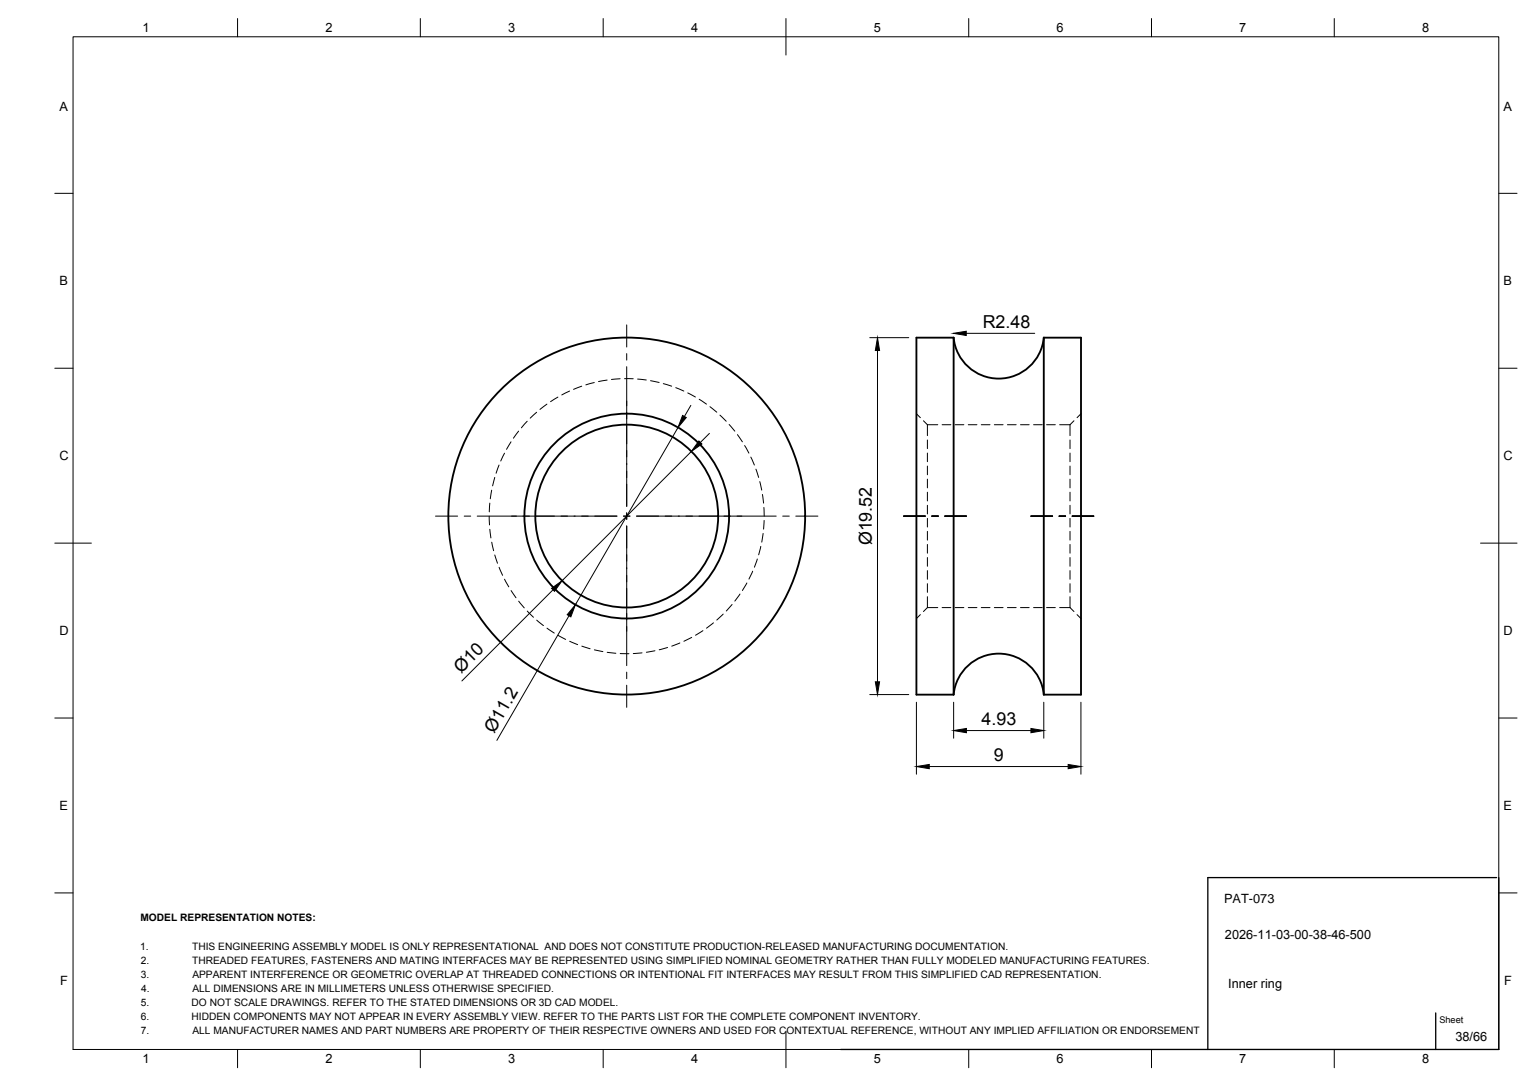
ISO-10303-21;
HEADER;
/* Generated by software containing ST-Developer
 * from STEP Tools, Inc. (www.steptools.com) 
 */

FILE_DESCRIPTION(
/* description */ ('Manual piston pump'),
/* implementation_level */ '2;1');

FILE_NAME(
/* name */ 'Inner ring.step',
/* time_stamp */ '2026-11-02T16:54:23-08:00',
/* author */ (''),
/* organization */ (''),
/* preprocessor_version */ 'ST-DEVELOPER v20.2',
/* originating_system */ 'Autodesk Translation Framework v15.17.0.0',
/* authorisation */ '');

FILE_SCHEMA (('AUTOMOTIVE_DESIGN { 1 0 10303 214 3 1 1 }'));
ENDSEC;

DATA;
#10=MECHANICAL_DESIGN_GEOMETRIC_PRESENTATION_REPRESENTATION('',(#711),#19043);
#537=CONICAL_SURFACE('',#10717,0.53,0.785398163397448);
#538=CONICAL_SURFACE('',#10724,0.53,0.785398163397448);
#559=TOROIDAL_SURFACE('',#10706,1.,0.247676);
#585=SHAPE_REPRESENTATION_RELATIONSHIP('SRR','None',#19332,#648);
#648=ADVANCED_BREP_SHAPE_REPRESENTATION('',(#781),#18999);
#711=STYLED_ITEM('',(#19664),#781);
#781=MANIFOLD_SOLID_BREP('Body1',#9497);
#946=FACE_BOUND('',#2229,.T.);
#947=FACE_BOUND('',#2232,.T.);
#1183=CYLINDRICAL_SURFACE('',#10712,0.976185);
#1184=CYLINDRICAL_SURFACE('',#10714,0.5);
#1185=CYLINDRICAL_SURFACE('',#10720,0.976185);
#1530=FACE_OUTER_BOUND('',#2224,.T.);
#1531=FACE_OUTER_BOUND('',#2225,.T.);
#1532=FACE_OUTER_BOUND('',#2226,.T.);
#1533=FACE_OUTER_BOUND('',#2227,.T.);
#1534=FACE_OUTER_BOUND('',#2228,.T.);
#1535=FACE_OUTER_BOUND('',#2230,.T.);
#1536=FACE_OUTER_BOUND('',#2231,.T.);
#1537=FACE_OUTER_BOUND('',#2233,.T.);
#2224=EDGE_LOOP('',(#7249,#7250,#7251,#7252,#7253,#7254));
#2225=EDGE_LOOP('',(#7255,#7256,#7257,#7258,#7259));
#2226=EDGE_LOOP('',(#7260,#7261,#7262,#7263));
#2227=EDGE_LOOP('',(#7264,#7265,#7266,#7267));
#2228=EDGE_LOOP('',(#7268));
#2229=EDGE_LOOP('',(#7269));
#2230=EDGE_LOOP('',(#7270,#7271,#7272,#7273,#7274));
#2231=EDGE_LOOP('',(#7275));
#2232=EDGE_LOOP('',(#7276));
#2233=EDGE_LOOP('',(#7277,#7278,#7279,#7280));
#2861=CIRCLE('',#10707,0.976185);
#2862=CIRCLE('',#10708,0.976185);
#2863=CIRCLE('',#10709,0.247676);
#2864=CIRCLE('',#10710,0.976185);
#2865=CIRCLE('',#10711,0.976185);
#2866=CIRCLE('',#10713,0.976185);
#2867=CIRCLE('',#10715,0.5);
#2868=CIRCLE('',#10716,0.5);
#2869=CIRCLE('',#10718,0.56);
#2870=CIRCLE('',#10721,0.976185);
#2871=CIRCLE('',#10723,0.56);
#3422=LINE('',#15764,#4026);
#3423=LINE('',#15770,#4027);
#3424=LINE('',#15774,#4028);
#3425=LINE('',#15780,#4029);
#3426=LINE('',#15785,#4030);
#4026=VECTOR('',#12710,0.976185);
#4027=VECTOR('',#12717,0.5);
#4028=VECTOR('',#12722,0.53);
#4029=VECTOR('',#12731,0.976185);
#4030=VECTOR('',#12738,0.53);
#4676=VERTEX_POINT('',#15753);
#4677=VERTEX_POINT('',#15754);
#4678=VERTEX_POINT('',#15757);
#4679=VERTEX_POINT('',#15759);
#4680=VERTEX_POINT('',#15763);
#4681=VERTEX_POINT('',#15767);
#4682=VERTEX_POINT('',#15769);
#4683=VERTEX_POINT('',#15773);
#4684=VERTEX_POINT('',#15778);
#4685=VERTEX_POINT('',#15782);
#5611=EDGE_CURVE('',#4676,#4677,#2861,.T.);
#5612=EDGE_CURVE('',#4677,#4676,#2862,.T.);
#5613=EDGE_CURVE('',#4677,#4678,#2863,.T.);
#5614=EDGE_CURVE('',#4679,#4678,#2864,.T.);
#5615=EDGE_CURVE('',#4678,#4679,#2865,.T.);
#5616=EDGE_CURVE('',#4679,#4680,#3422,.T.);
#5617=EDGE_CURVE('',#4680,#4680,#2866,.T.);
#5618=EDGE_CURVE('',#4681,#4681,#2867,.T.);
#5619=EDGE_CURVE('',#4681,#4682,#3423,.T.);
#5620=EDGE_CURVE('',#4682,#4682,#2868,.T.);
#5621=EDGE_CURVE('',#4682,#4683,#3424,.T.);
#5622=EDGE_CURVE('',#4683,#4683,#2869,.T.);
#5623=EDGE_CURVE('',#4684,#4684,#2870,.T.);
#5624=EDGE_CURVE('',#4684,#4676,#3425,.T.);
#5625=EDGE_CURVE('',#4685,#4685,#2871,.T.);
#5626=EDGE_CURVE('',#4685,#4681,#3426,.T.);
#7249=ORIENTED_EDGE('',*,*,#5611,.F.);
#7250=ORIENTED_EDGE('',*,*,#5612,.F.);
#7251=ORIENTED_EDGE('',*,*,#5613,.T.);
#7252=ORIENTED_EDGE('',*,*,#5614,.F.);
#7253=ORIENTED_EDGE('',*,*,#5615,.F.);
#7254=ORIENTED_EDGE('',*,*,#5613,.F.);
#7255=ORIENTED_EDGE('',*,*,#5614,.T.);
#7256=ORIENTED_EDGE('',*,*,#5615,.T.);
#7257=ORIENTED_EDGE('',*,*,#5616,.T.);
#7258=ORIENTED_EDGE('',*,*,#5617,.T.);
#7259=ORIENTED_EDGE('',*,*,#5616,.F.);
#7260=ORIENTED_EDGE('',*,*,#5618,.T.);
#7261=ORIENTED_EDGE('',*,*,#5619,.T.);
#7262=ORIENTED_EDGE('',*,*,#5620,.F.);
#7263=ORIENTED_EDGE('',*,*,#5619,.F.);
#7264=ORIENTED_EDGE('',*,*,#5620,.T.);
#7265=ORIENTED_EDGE('',*,*,#5621,.T.);
#7266=ORIENTED_EDGE('',*,*,#5622,.F.);
#7267=ORIENTED_EDGE('',*,*,#5621,.F.);
#7268=ORIENTED_EDGE('',*,*,#5617,.F.);
#7269=ORIENTED_EDGE('',*,*,#5622,.T.);
#7270=ORIENTED_EDGE('',*,*,#5623,.F.);
#7271=ORIENTED_EDGE('',*,*,#5624,.T.);
#7272=ORIENTED_EDGE('',*,*,#5611,.T.);
#7273=ORIENTED_EDGE('',*,*,#5612,.T.);
#7274=ORIENTED_EDGE('',*,*,#5624,.F.);
#7275=ORIENTED_EDGE('',*,*,#5623,.T.);
#7276=ORIENTED_EDGE('',*,*,#5625,.F.);
#7277=ORIENTED_EDGE('',*,*,#5625,.T.);
#7278=ORIENTED_EDGE('',*,*,#5626,.T.);
#7279=ORIENTED_EDGE('',*,*,#5618,.F.);
#7280=ORIENTED_EDGE('',*,*,#5626,.F.);
#8708=PLANE('',#10719);
#8709=PLANE('',#10722);
#9135=ADVANCED_FACE('',(#1530),#559,.F.);
#9136=ADVANCED_FACE('',(#1531),#1183,.T.);
#9137=ADVANCED_FACE('',(#1532),#1184,.F.);
#9138=ADVANCED_FACE('',(#1533),#537,.F.);
#9139=ADVANCED_FACE('',(#1534,#946),#8708,.T.);
#9140=ADVANCED_FACE('',(#1535),#1185,.T.);
#9141=ADVANCED_FACE('',(#1536,#947),#8709,.T.);
#9142=ADVANCED_FACE('',(#1537),#538,.F.);
#9497=CLOSED_SHELL('',(#9135,#9136,#9137,#9138,#9139,#9140,#9141,#9142));
#10705=AXIS2_PLACEMENT_3D('',#15751,#12694,#12695);
#10706=AXIS2_PLACEMENT_3D('',#15752,#12696,#12697);
#10707=AXIS2_PLACEMENT_3D('',#15755,#12698,#12699);
#10708=AXIS2_PLACEMENT_3D('',#15756,#12700,#12701);
#10709=AXIS2_PLACEMENT_3D('',#15758,#12702,#12703);
#10710=AXIS2_PLACEMENT_3D('',#15760,#12704,#12705);
#10711=AXIS2_PLACEMENT_3D('',#15761,#12706,#12707);
#10712=AXIS2_PLACEMENT_3D('',#15762,#12708,#12709);
#10713=AXIS2_PLACEMENT_3D('',#15765,#12711,#12712);
#10714=AXIS2_PLACEMENT_3D('',#15766,#12713,#12714);
#10715=AXIS2_PLACEMENT_3D('',#15768,#12715,#12716);
#10716=AXIS2_PLACEMENT_3D('',#15771,#12718,#12719);
#10717=AXIS2_PLACEMENT_3D('',#15772,#12720,#12721);
#10718=AXIS2_PLACEMENT_3D('',#15775,#12723,#12724);
#10719=AXIS2_PLACEMENT_3D('',#15776,#12725,#12726);
#10720=AXIS2_PLACEMENT_3D('',#15777,#12727,#12728);
#10721=AXIS2_PLACEMENT_3D('',#15779,#12729,#12730);
#10722=AXIS2_PLACEMENT_3D('',#15781,#12732,#12733);
#10723=AXIS2_PLACEMENT_3D('',#15783,#12734,#12735);
#10724=AXIS2_PLACEMENT_3D('',#15784,#12736,#12737);
#12694=DIRECTION('axis',(0.,0.,1.));
#12695=DIRECTION('refdir',(1.,0.,0.));
#12696=DIRECTION('center_axis',(0.,-1.,0.));
#12697=DIRECTION('ref_axis',(0.,0.,-1.));
#12698=DIRECTION('center_axis',(0.,-1.,0.));
#12699=DIRECTION('ref_axis',(1.,0.,0.));
#12700=DIRECTION('center_axis',(0.,-1.,0.));
#12701=DIRECTION('ref_axis',(1.,0.,0.));
#12702=DIRECTION('center_axis',(1.,0.,1.22464679914735E-16));
#12703=DIRECTION('ref_axis',(-1.22464679914735E-16,0.,1.));
#12704=DIRECTION('center_axis',(0.,1.,0.));
#12705=DIRECTION('ref_axis',(1.,0.,0.));
#12706=DIRECTION('center_axis',(0.,1.,0.));
#12707=DIRECTION('ref_axis',(1.,0.,0.));
#12708=DIRECTION('center_axis',(0.,-1.,0.));
#12709=DIRECTION('ref_axis',(1.,0.,0.));
#12710=DIRECTION('',(0.,1.,0.));
#12711=DIRECTION('center_axis',(0.,-1.,0.));
#12712=DIRECTION('ref_axis',(1.,0.,0.));
#12713=DIRECTION('center_axis',(0.,-1.,0.));
#12714=DIRECTION('ref_axis',(1.,0.,0.));
#12715=DIRECTION('center_axis',(0.,-1.,0.));
#12716=DIRECTION('ref_axis',(1.,0.,0.));
#12717=DIRECTION('',(0.,1.,0.));
#12718=DIRECTION('center_axis',(0.,-1.,0.));
#12719=DIRECTION('ref_axis',(1.,0.,0.));
#12720=DIRECTION('center_axis',(0.,1.,0.));
#12721=DIRECTION('ref_axis',(1.,0.,0.));
#12722=DIRECTION('',(-0.707106781186547,0.707106781186548,-8.65956056235493E-17));
#12723=DIRECTION('center_axis',(0.,-1.,0.));
#12724=DIRECTION('ref_axis',(1.,0.,0.));
#12725=DIRECTION('center_axis',(0.,1.,0.));
#12726=DIRECTION('ref_axis',(0.,0.,1.));
#12727=DIRECTION('center_axis',(0.,-1.,0.));
#12728=DIRECTION('ref_axis',(1.,0.,0.));
#12729=DIRECTION('center_axis',(0.,-1.,0.));
#12730=DIRECTION('ref_axis',(1.,0.,0.));
#12731=DIRECTION('',(0.,1.,0.));
#12732=DIRECTION('center_axis',(0.,-1.,0.));
#12733=DIRECTION('ref_axis',(0.,0.,-1.));
#12734=DIRECTION('center_axis',(0.,-1.,0.));
#12735=DIRECTION('ref_axis',(1.,0.,0.));
#12736=DIRECTION('center_axis',(0.,-1.,0.));
#12737=DIRECTION('ref_axis',(1.,0.,0.));
#12738=DIRECTION('',(0.707106781186547,0.707106781186548,8.65956056235493E-17));
#15751=CARTESIAN_POINT('',(0.,0.,0.));
#15752=CARTESIAN_POINT('Origin',(0.,0.,0.));
#15753=CARTESIAN_POINT('',(-0.976185,-0.246528389340863,-1.19548183562566E-16));
#15754=CARTESIAN_POINT('',(-1.19548183562566E-16,-0.246528389340863,0.976185));
#15755=CARTESIAN_POINT('Origin',(0.,-0.246528389340863,0.));
#15756=CARTESIAN_POINT('Origin',(0.,-0.246528389340863,0.));
#15757=CARTESIAN_POINT('',(-1.19548183562566E-16,0.246528389340863,0.976185));
#15758=CARTESIAN_POINT('Origin',(-1.22464679914735E-16,0.,1.));
#15759=CARTESIAN_POINT('',(-0.976185,0.246528389340863,1.19548183562566E-16));
#15760=CARTESIAN_POINT('Origin',(0.,0.246528389340863,0.));
#15761=CARTESIAN_POINT('Origin',(0.,0.246528389340863,0.));
#15762=CARTESIAN_POINT('Origin',(0.,0.,0.));
#15763=CARTESIAN_POINT('',(-0.976185,0.45,-1.19548183562566E-16));
#15764=CARTESIAN_POINT('',(-0.976185,0.,-1.19548183562566E-16));
#15765=CARTESIAN_POINT('Origin',(0.,0.45,0.));
#15766=CARTESIAN_POINT('Origin',(0.,0.,0.));
#15767=CARTESIAN_POINT('',(-0.5,-0.39,-6.12323399573677E-17));
#15768=CARTESIAN_POINT('Origin',(0.,-0.39,0.));
#15769=CARTESIAN_POINT('',(-0.5,0.39,-6.12323399573677E-17));
#15770=CARTESIAN_POINT('',(-0.5,0.,-6.12323399573677E-17));
#15771=CARTESIAN_POINT('Origin',(0.,0.39,0.));
#15772=CARTESIAN_POINT('Origin',(0.,0.42,0.));
#15773=CARTESIAN_POINT('',(-0.56,0.45,-6.85802207522518E-17));
#15774=CARTESIAN_POINT('',(-0.53,0.42,-6.49062803548097E-17));
#15775=CARTESIAN_POINT('Origin',(0.,0.45,0.));
#15776=CARTESIAN_POINT('Origin',(0.976185,0.45,0.));
#15777=CARTESIAN_POINT('Origin',(0.,0.,0.));
#15778=CARTESIAN_POINT('',(-0.976185,-0.45,-1.19548183562566E-16));
#15779=CARTESIAN_POINT('Origin',(0.,-0.45,0.));
#15780=CARTESIAN_POINT('',(-0.976185,0.,-1.19548183562566E-16));
#15781=CARTESIAN_POINT('Origin',(0.56,-0.45,0.));
#15782=CARTESIAN_POINT('',(-0.56,-0.45,-6.85802207522518E-17));
#15783=CARTESIAN_POINT('Origin',(0.,-0.45,0.));
#15784=CARTESIAN_POINT('Origin',(0.,-0.42,0.));
#15785=CARTESIAN_POINT('',(-0.53,-0.42,-6.49062803548097E-17));
#18928=UNCERTAINTY_MEASURE_WITH_UNIT(LENGTH_MEASURE(0.001),#19044,
'DISTANCE_ACCURACY_VALUE',
'Maximum model space distance between geometric entities at asserted c
onnectivities');
#18972=UNCERTAINTY_MEASURE_WITH_UNIT(LENGTH_MEASURE(0.001),#19044,
'DISTANCE_ACCURACY_VALUE',
'Maximum model space distance between geometric entities at asserted c
onnectivities');
#18999=(
GEOMETRIC_REPRESENTATION_CONTEXT(3)
GLOBAL_UNCERTAINTY_ASSIGNED_CONTEXT((#18928))
GLOBAL_UNIT_ASSIGNED_CONTEXT((#19044,#19046,#19047))
REPRESENTATION_CONTEXT('','3D')
);
#19043=(
GEOMETRIC_REPRESENTATION_CONTEXT(3)
GLOBAL_UNCERTAINTY_ASSIGNED_CONTEXT((#18972))
GLOBAL_UNIT_ASSIGNED_CONTEXT((#19044,#19046,#19047))
REPRESENTATION_CONTEXT('','3D')
);
#19044=(
LENGTH_UNIT()
NAMED_UNIT(*)
SI_UNIT(.CENTI.,.METRE.)
);
#19046=(
NAMED_UNIT(*)
PLANE_ANGLE_UNIT()
SI_UNIT($,.RADIAN.)
);
#19047=(
NAMED_UNIT(*)
SI_UNIT($,.STERADIAN.)
SOLID_ANGLE_UNIT()
);
#19074=SHAPE_DEFINITION_REPRESENTATION(#19144,#19332);
#19144=PRODUCT_DEFINITION_SHAPE('',$,#19403);
#19332=SHAPE_REPRESENTATION('',(#10705),#18999);
#19376=PRODUCT_DEFINITION_CONTEXT('part definition',#19588,'design');
#19403=PRODUCT_DEFINITION('2026-11-03-00-38-46-500','Inner ring',#19473,
#19376);
#19473=PRODUCT_DEFINITION_FORMATION('',$,#19616);
#19588=APPLICATION_CONTEXT(
'Core Data for Automotive Mechanical Design Process');
#19589=PRODUCT_CONTEXT('part definition',#19588,'mechanical');
#19616=PRODUCT('2026-11-03-00-38-46-500','Inner ring','Inner ring',(#19589));
#19664=PRESENTATION_STYLE_ASSIGNMENT((#19670));
#19670=SURFACE_STYLE_USAGE(.BOTH.,#19676);
#19676=SURFACE_SIDE_STYLE('',(#19682));
#19682=SURFACE_STYLE_FILL_AREA(#19688);
#19688=FILL_AREA_STYLE('CAD Library Painted - Steel gray',(#19694));
#19694=FILL_AREA_STYLE_COLOUR('CAD Library Painted - Steel gray',#19700);
#19700=COLOUR_RGB('CAD Library Painted - Steel gray',0.592156862745098,
0.631372549019608,0.67843137254902);
ENDSEC;
END-ISO-10303-21;
